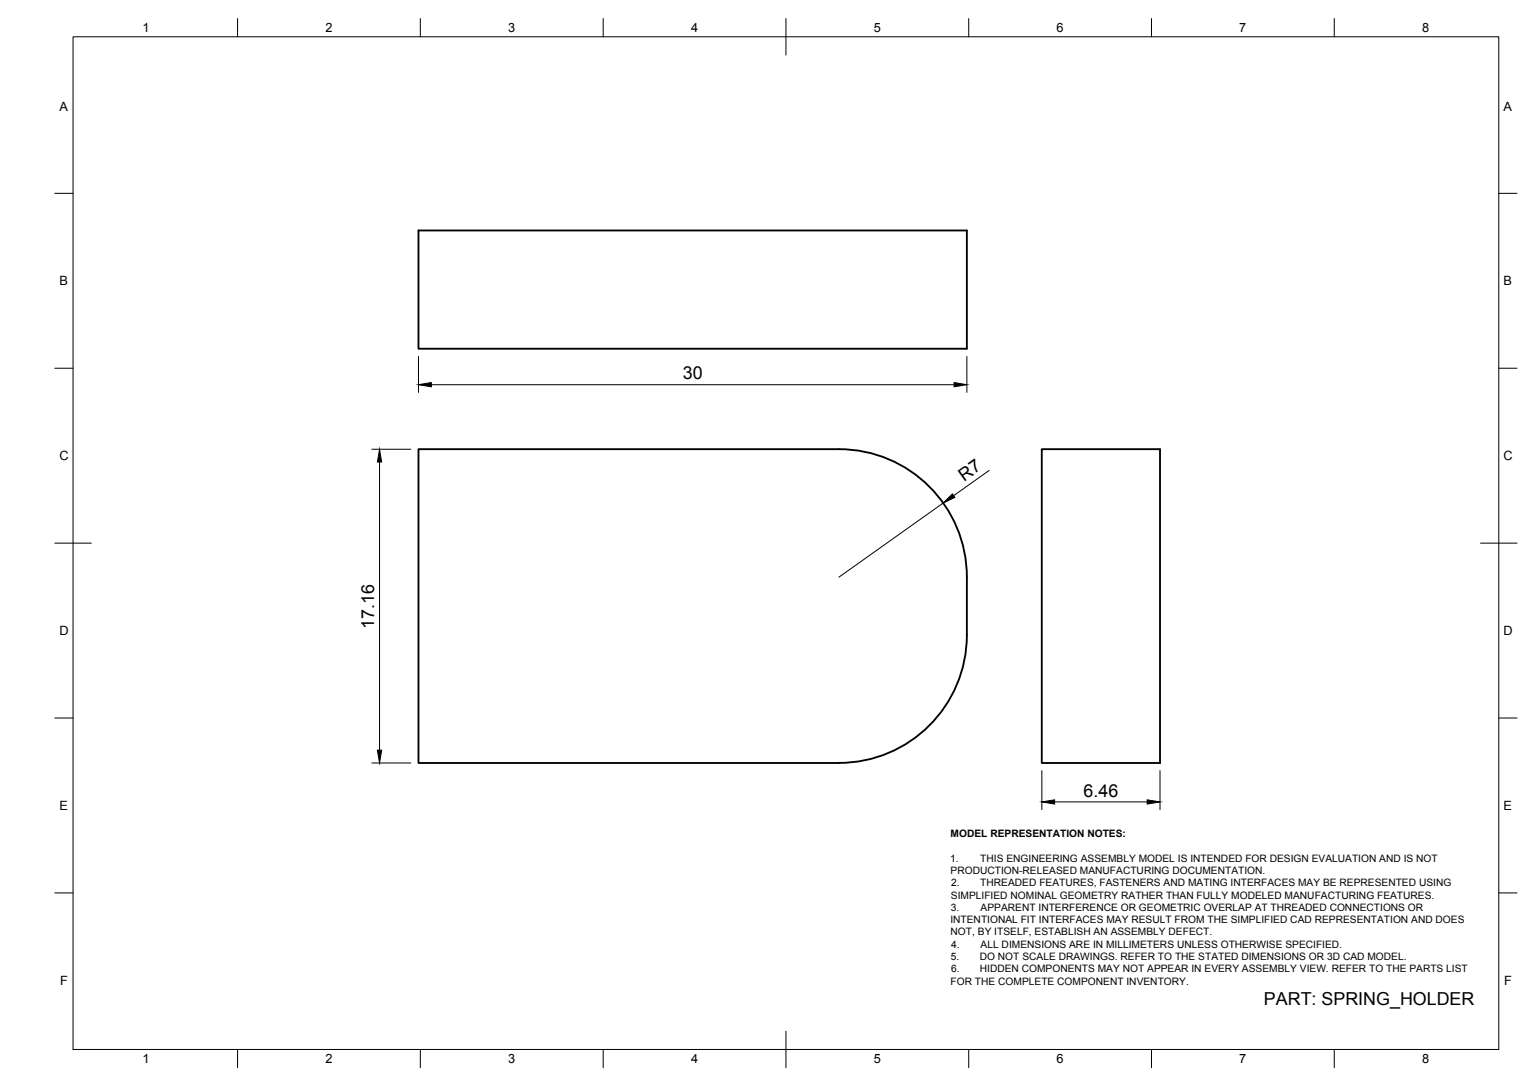
ISO-10303-21;
HEADER;
/* Generated by software containing ST-Developer
 * from STEP Tools, Inc. (www.steptools.com) 
 */

FILE_DESCRIPTION(
/* description */ (''),
/* implementation_level */ '2;1');

FILE_NAME(
/* name */ 'Spring_Holder.step',
/* time_stamp */ '2026-09-20T22:38:01+06:00',
/* author */ (''),
/* organization */ (''),
/* preprocessor_version */ 'ST-DEVELOPER v20.2',
/* originating_system */ 'Autodesk Translation Framework v15.15.0.0',
/* authorisation */ '');

FILE_SCHEMA (('AUTOMOTIVE_DESIGN { 1 0 10303 214 3 1 1 }'));
ENDSEC;

DATA;
#10=MECHANICAL_DESIGN_GEOMETRIC_PRESENTATION_REPRESENTATION('',(#89),#4079);
#73=SHAPE_REPRESENTATION_RELATIONSHIP('SRR','None',#4116,#81);
#81=ADVANCED_BREP_SHAPE_REPRESENTATION('',(#97),#4076);
#89=STYLED_ITEM('',(#4159),#97);
#97=MANIFOLD_SOLID_BREP('Spring_Holder',#1448);
#163=CIRCLE('',#1666,7.);
#164=CIRCLE('',#1667,7.);
#165=CIRCLE('',#1670,7.);
#166=CIRCLE('',#1672,7.);
#194=CYLINDRICAL_SURFACE('',#1665,7.);
#195=CYLINDRICAL_SURFACE('',#1671,7.);
#264=FACE_OUTER_BOUND('',#354,.T.);
#265=FACE_OUTER_BOUND('',#355,.T.);
#266=FACE_OUTER_BOUND('',#356,.T.);
#267=FACE_OUTER_BOUND('',#357,.T.);
#268=FACE_OUTER_BOUND('',#358,.T.);
#269=FACE_OUTER_BOUND('',#359,.T.);
#270=FACE_OUTER_BOUND('',#360,.T.);
#271=FACE_OUTER_BOUND('',#361,.T.);
#354=EDGE_LOOP('',(#1243,#1244,#1245,#1246));
#355=EDGE_LOOP('',(#1247,#1248,#1249,#1250));
#356=EDGE_LOOP('',(#1251,#1252,#1253,#1254,#1255,#1256));
#357=EDGE_LOOP('',(#1257,#1258,#1259,#1260));
#358=EDGE_LOOP('',(#1261,#1262,#1263,#1264,#1265,#1266));
#359=EDGE_LOOP('',(#1267,#1268,#1269,#1270));
#360=EDGE_LOOP('',(#1271,#1272,#1273,#1274));
#361=EDGE_LOOP('',(#1275,#1276,#1277,#1278));
#457=LINE('',#3983,#570);
#458=LINE('',#3986,#571);
#459=LINE('',#3989,#572);
#460=LINE('',#3991,#573);
#461=LINE('',#3992,#574);
#462=LINE('',#3995,#575);
#463=LINE('',#3997,#576);
#464=LINE('',#3999,#577);
#465=LINE('',#4004,#578);
#466=LINE('',#4007,#579);
#467=LINE('',#4009,#580);
#468=LINE('',#4010,#581);
#469=LINE('',#4012,#582);
#470=LINE('',#4014,#583);
#570=VECTOR('',#2038,10.);
#571=VECTOR('',#2041,10.);
#572=VECTOR('',#2044,10.);
#573=VECTOR('',#2045,10.);
#574=VECTOR('',#2046,10.);
#575=VECTOR('',#2049,10.);
#576=VECTOR('',#2050,10.);
#577=VECTOR('',#2051,10.);
#578=VECTOR('',#2058,10.);
#579=VECTOR('',#2061,10.);
#580=VECTOR('',#2062,10.);
#581=VECTOR('',#2063,10.);
#582=VECTOR('',#2066,10.);
#583=VECTOR('',#2069,10.);
#702=VERTEX_POINT('',#3979);
#703=VERTEX_POINT('',#3980);
#704=VERTEX_POINT('',#3982);
#705=VERTEX_POINT('',#3984);
#706=VERTEX_POINT('',#3988);
#707=VERTEX_POINT('',#3990);
#708=VERTEX_POINT('',#3994);
#709=VERTEX_POINT('',#3996);
#710=VERTEX_POINT('',#3998);
#711=VERTEX_POINT('',#4002);
#712=VERTEX_POINT('',#4006);
#713=VERTEX_POINT('',#4008);
#886=EDGE_CURVE('',#702,#703,#163,.T.);
#887=EDGE_CURVE('',#703,#704,#457,.T.);
#888=EDGE_CURVE('',#704,#705,#164,.T.);
#889=EDGE_CURVE('',#705,#702,#458,.T.);
#890=EDGE_CURVE('',#703,#706,#459,.T.);
#891=EDGE_CURVE('',#707,#706,#460,.T.);
#892=EDGE_CURVE('',#707,#704,#461,.T.);
#893=EDGE_CURVE('',#708,#702,#462,.T.);
#894=EDGE_CURVE('',#709,#708,#463,.T.);
#895=EDGE_CURVE('',#709,#710,#464,.T.);
#896=EDGE_CURVE('',#706,#710,#165,.T.);
#897=EDGE_CURVE('',#711,#707,#166,.T.);
#898=EDGE_CURVE('',#710,#711,#465,.T.);
#899=EDGE_CURVE('',#712,#711,#466,.T.);
#900=EDGE_CURVE('',#713,#712,#467,.T.);
#901=EDGE_CURVE('',#713,#705,#468,.T.);
#902=EDGE_CURVE('',#712,#709,#469,.T.);
#903=EDGE_CURVE('',#708,#713,#470,.T.);
#1243=ORIENTED_EDGE('',*,*,#886,.T.);
#1244=ORIENTED_EDGE('',*,*,#887,.T.);
#1245=ORIENTED_EDGE('',*,*,#888,.T.);
#1246=ORIENTED_EDGE('',*,*,#889,.T.);
#1247=ORIENTED_EDGE('',*,*,#887,.F.);
#1248=ORIENTED_EDGE('',*,*,#890,.T.);
#1249=ORIENTED_EDGE('',*,*,#891,.F.);
#1250=ORIENTED_EDGE('',*,*,#892,.T.);
#1251=ORIENTED_EDGE('',*,*,#886,.F.);
#1252=ORIENTED_EDGE('',*,*,#893,.F.);
#1253=ORIENTED_EDGE('',*,*,#894,.F.);
#1254=ORIENTED_EDGE('',*,*,#895,.T.);
#1255=ORIENTED_EDGE('',*,*,#896,.F.);
#1256=ORIENTED_EDGE('',*,*,#890,.F.);
#1257=ORIENTED_EDGE('',*,*,#897,.T.);
#1258=ORIENTED_EDGE('',*,*,#891,.T.);
#1259=ORIENTED_EDGE('',*,*,#896,.T.);
#1260=ORIENTED_EDGE('',*,*,#898,.T.);
#1261=ORIENTED_EDGE('',*,*,#888,.F.);
#1262=ORIENTED_EDGE('',*,*,#892,.F.);
#1263=ORIENTED_EDGE('',*,*,#897,.F.);
#1264=ORIENTED_EDGE('',*,*,#899,.F.);
#1265=ORIENTED_EDGE('',*,*,#900,.F.);
#1266=ORIENTED_EDGE('',*,*,#901,.T.);
#1267=ORIENTED_EDGE('',*,*,#898,.F.);
#1268=ORIENTED_EDGE('',*,*,#895,.F.);
#1269=ORIENTED_EDGE('',*,*,#902,.F.);
#1270=ORIENTED_EDGE('',*,*,#899,.T.);
#1271=ORIENTED_EDGE('',*,*,#889,.F.);
#1272=ORIENTED_EDGE('',*,*,#901,.F.);
#1273=ORIENTED_EDGE('',*,*,#903,.F.);
#1274=ORIENTED_EDGE('',*,*,#893,.T.);
#1275=ORIENTED_EDGE('',*,*,#900,.T.);
#1276=ORIENTED_EDGE('',*,*,#902,.T.);
#1277=ORIENTED_EDGE('',*,*,#894,.T.);
#1278=ORIENTED_EDGE('',*,*,#903,.T.);
#1345=PLANE('',#1668);
#1346=PLANE('',#1669);
#1347=PLANE('',#1673);
#1348=PLANE('',#1674);
#1349=PLANE('',#1675);
#1350=PLANE('',#1676);
#1426=ADVANCED_FACE('',(#264),#194,.T.);
#1427=ADVANCED_FACE('',(#265),#1345,.T.);
#1428=ADVANCED_FACE('',(#266),#1346,.T.);
#1429=ADVANCED_FACE('',(#267),#195,.T.);
#1430=ADVANCED_FACE('',(#268),#1347,.T.);
#1431=ADVANCED_FACE('',(#269),#1348,.T.);
#1432=ADVANCED_FACE('',(#270),#1349,.T.);
#1433=ADVANCED_FACE('',(#271),#1350,.F.);
#1448=CLOSED_SHELL('',(#1426,#1427,#1428,#1429,#1430,#1431,#1432,#1433));
#1664=AXIS2_PLACEMENT_3D('',#3977,#2032,#2033);
#1665=AXIS2_PLACEMENT_3D('',#3978,#2034,#2035);
#1666=AXIS2_PLACEMENT_3D('',#3981,#2036,#2037);
#1667=AXIS2_PLACEMENT_3D('',#3985,#2039,#2040);
#1668=AXIS2_PLACEMENT_3D('',#3987,#2042,#2043);
#1669=AXIS2_PLACEMENT_3D('',#3993,#2047,#2048);
#1670=AXIS2_PLACEMENT_3D('',#4000,#2052,#2053);
#1671=AXIS2_PLACEMENT_3D('',#4001,#2054,#2055);
#1672=AXIS2_PLACEMENT_3D('',#4003,#2056,#2057);
#1673=AXIS2_PLACEMENT_3D('',#4005,#2059,#2060);
#1674=AXIS2_PLACEMENT_3D('',#4011,#2064,#2065);
#1675=AXIS2_PLACEMENT_3D('',#4013,#2067,#2068);
#1676=AXIS2_PLACEMENT_3D('',#4015,#2070,#2071);
#2032=DIRECTION('axis',(0.,0.,1.));
#2033=DIRECTION('refdir',(1.,0.,0.));
#2034=DIRECTION('center_axis',(0.,0.,1.));
#2035=DIRECTION('ref_axis',(0.707106781186548,-0.707106781186547,0.));
#2036=DIRECTION('center_axis',(0.,0.,-1.));
#2037=DIRECTION('ref_axis',(0.707106781186548,-0.707106781186547,0.));
#2038=DIRECTION('',(0.,0.,-1.));
#2039=DIRECTION('center_axis',(0.,0.,1.));
#2040=DIRECTION('ref_axis',(0.707106781186548,-0.707106781186547,0.));
#2041=DIRECTION('',(0.,0.,1.));
#2042=DIRECTION('center_axis',(0.,-1.,0.));
#2043=DIRECTION('ref_axis',(0.,0.,-1.));
#2044=DIRECTION('',(-1.,0.,0.));
#2045=DIRECTION('',(0.,0.,1.));
#2046=DIRECTION('',(1.,0.,0.));
#2047=DIRECTION('center_axis',(0.,0.,1.));
#2048=DIRECTION('ref_axis',(-1.,0.,0.));
#2049=DIRECTION('',(0.,-1.,0.));
#2050=DIRECTION('',(1.,0.,0.));
#2051=DIRECTION('',(0.,-1.,0.));
#2052=DIRECTION('center_axis',(0.,0.,-1.));
#2053=DIRECTION('ref_axis',(-0.707106781186548,-0.707106781186547,0.));
#2054=DIRECTION('center_axis',(0.,0.,-1.));
#2055=DIRECTION('ref_axis',(-0.707106781186548,-0.707106781186547,0.));
#2056=DIRECTION('center_axis',(0.,0.,1.));
#2057=DIRECTION('ref_axis',(-0.707106781186548,-0.707106781186547,0.));
#2058=DIRECTION('',(0.,0.,-1.));
#2059=DIRECTION('center_axis',(0.,0.,-1.));
#2060=DIRECTION('ref_axis',(1.,0.,0.));
#2061=DIRECTION('',(0.,-1.,0.));
#2062=DIRECTION('',(-1.,0.,0.));
#2063=DIRECTION('',(0.,-1.,0.));
#2064=DIRECTION('center_axis',(-1.,0.,0.));
#2065=DIRECTION('ref_axis',(0.,0.,-1.));
#2066=DIRECTION('',(0.,0.,1.));
#2067=DIRECTION('center_axis',(1.,0.,0.));
#2068=DIRECTION('ref_axis',(0.,0.,1.));
#2069=DIRECTION('',(0.,0.,-1.));
#2070=DIRECTION('center_axis',(0.,-1.,0.));
#2071=DIRECTION('ref_axis',(1.,0.,0.));
#3977=CARTESIAN_POINT('',(0.,0.,0.));
#3978=CARTESIAN_POINT('Origin',(59.5698926278372,-18.,39.6167831756372));
#3979=CARTESIAN_POINT('',(66.5698926278372,-18.,44.4641879853147));
#3980=CARTESIAN_POINT('',(59.5698926278372,-25.,44.4641879853147));
#3981=CARTESIAN_POINT('Origin',(59.5698926278372,-18.,44.4641879853147));
#3982=CARTESIAN_POINT('',(59.5698926278372,-25.,38.0009815724114));
#3983=CARTESIAN_POINT('',(59.5698926278372,-25.,39.6167831756372));
#3984=CARTESIAN_POINT('',(66.5698926278372,-18.,38.0009815724114));
#3985=CARTESIAN_POINT('Origin',(59.5698926278372,-18.,38.0009815724114));
#3986=CARTESIAN_POINT('',(66.5698926278372,-18.,39.6167831756372));
#3987=CARTESIAN_POINT('Origin',(57.9894289417414,-25.,41.2325847788631));
#3988=CARTESIAN_POINT('',(56.4089652556457,-25.,44.4641879853147));
#3989=CARTESIAN_POINT('',(49.4089652556457,-25.,44.4641879853147));
#3990=CARTESIAN_POINT('',(56.4089652556457,-25.,38.0009815724114));
#3991=CARTESIAN_POINT('',(56.4089652556457,-25.,42.8483863820889));
#3992=CARTESIAN_POINT('',(66.5698926278372,-25.,38.0009815724114));
#3993=CARTESIAN_POINT('Origin',(66.5698926278372,5.,44.4641879853147));
#3994=CARTESIAN_POINT('',(66.5698926278372,5.,44.4641879853147));
#3995=CARTESIAN_POINT('',(66.5698926278372,5.,44.4641879853147));
#3996=CARTESIAN_POINT('',(49.4089652556457,5.,44.4641879853147));
#3997=CARTESIAN_POINT('',(49.4089652556457,5.,44.4641879853147));
#3998=CARTESIAN_POINT('',(49.4089652556457,-18.,44.4641879853147));
#3999=CARTESIAN_POINT('',(49.4089652556457,5.,44.4641879853147));
#4000=CARTESIAN_POINT('Origin',(56.4089652556457,-18.,44.4641879853147));
#4001=CARTESIAN_POINT('Origin',(56.4089652556457,-18.,42.8483863820889));
#4002=CARTESIAN_POINT('',(49.4089652556457,-18.,38.0009815724114));
#4003=CARTESIAN_POINT('Origin',(56.4089652556457,-18.,38.0009815724114));
#4004=CARTESIAN_POINT('',(49.4089652556457,-18.,42.8483863820889));
#4005=CARTESIAN_POINT('Origin',(49.4089652556457,5.,38.0009815724114));
#4006=CARTESIAN_POINT('',(49.4089652556457,5.,38.0009815724114));
#4007=CARTESIAN_POINT('',(49.4089652556457,5.,38.0009815724114));
#4008=CARTESIAN_POINT('',(66.5698926278372,5.,38.0009815724114));
#4009=CARTESIAN_POINT('',(66.5698926278372,5.,38.0009815724114));
#4010=CARTESIAN_POINT('',(66.5698926278372,5.,38.0009815724114));
#4011=CARTESIAN_POINT('Origin',(49.4089652556457,5.,44.4641879853147));
#4012=CARTESIAN_POINT('',(49.4089652556457,5.,38.0009815724114));
#4013=CARTESIAN_POINT('Origin',(66.5698926278372,5.,38.0009815724114));
#4014=CARTESIAN_POINT('',(66.5698926278372,5.,44.4641879853147));
#4015=CARTESIAN_POINT('Origin',(57.9894289417414,5.,41.2325847788631));
#4066=UNCERTAINTY_MEASURE_WITH_UNIT(LENGTH_MEASURE(0.01),#4080,
'DISTANCE_ACCURACY_VALUE',
'Maximum model space distance between geometric entities at asserted c
onnectivities');
#4069=UNCERTAINTY_MEASURE_WITH_UNIT(LENGTH_MEASURE(0.01),#4080,
'DISTANCE_ACCURACY_VALUE',
'Maximum model space distance between geometric entities at asserted c
onnectivities');
#4076=(
GEOMETRIC_REPRESENTATION_CONTEXT(3)
GLOBAL_UNCERTAINTY_ASSIGNED_CONTEXT((#4066))
GLOBAL_UNIT_ASSIGNED_CONTEXT((#4080,#4082,#4083))
REPRESENTATION_CONTEXT('','3D')
);
#4079=(
GEOMETRIC_REPRESENTATION_CONTEXT(3)
GLOBAL_UNCERTAINTY_ASSIGNED_CONTEXT((#4069))
GLOBAL_UNIT_ASSIGNED_CONTEXT((#4080,#4082,#4083))
REPRESENTATION_CONTEXT('','3D')
);
#4080=(
LENGTH_UNIT()
NAMED_UNIT(*)
SI_UNIT(.MILLI.,.METRE.)
);
#4082=(
NAMED_UNIT(*)
PLANE_ANGLE_UNIT()
SI_UNIT($,.RADIAN.)
);
#4083=(
NAMED_UNIT(*)
SI_UNIT($,.STERADIAN.)
SOLID_ANGLE_UNIT()
);
#4090=SHAPE_DEFINITION_REPRESENTATION(#4099,#4116);
#4099=PRODUCT_DEFINITION_SHAPE('',$,#4126);
#4116=SHAPE_REPRESENTATION('',(#1664),#4076);
#4119=PRODUCT_DEFINITION_CONTEXT('part definition',#4148,'design');
#4126=PRODUCT_DEFINITION('Spring_Holder','Spring_Holder',#4135,#4119);
#4135=PRODUCT_DEFINITION_FORMATION('',$,#4156);
#4148=APPLICATION_CONTEXT(
'Core Data for Automotive Mechanical Design Process');
#4149=PRODUCT_CONTEXT('part definition',#4148,'mechanical');
#4156=PRODUCT('Spring_Holder','Spring_Holder',$,(#4149));
#4159=PRESENTATION_STYLE_ASSIGNMENT((#4163));
#4163=SURFACE_STYLE_USAGE(.BOTH.,#4167);
#4167=SURFACE_SIDE_STYLE('',(#4171));
#4171=SURFACE_STYLE_FILL_AREA(#4175);
#4175=FILL_AREA_STYLE('Steel - Satin',(#4179));
#4179=FILL_AREA_STYLE_COLOUR('Steel - Satin',#4183);
#4183=COLOUR_RGB('Steel - Satin', 0.40784314, 0.44705882, 0.49803922);
ENDSEC;
END-ISO-10303-21;
